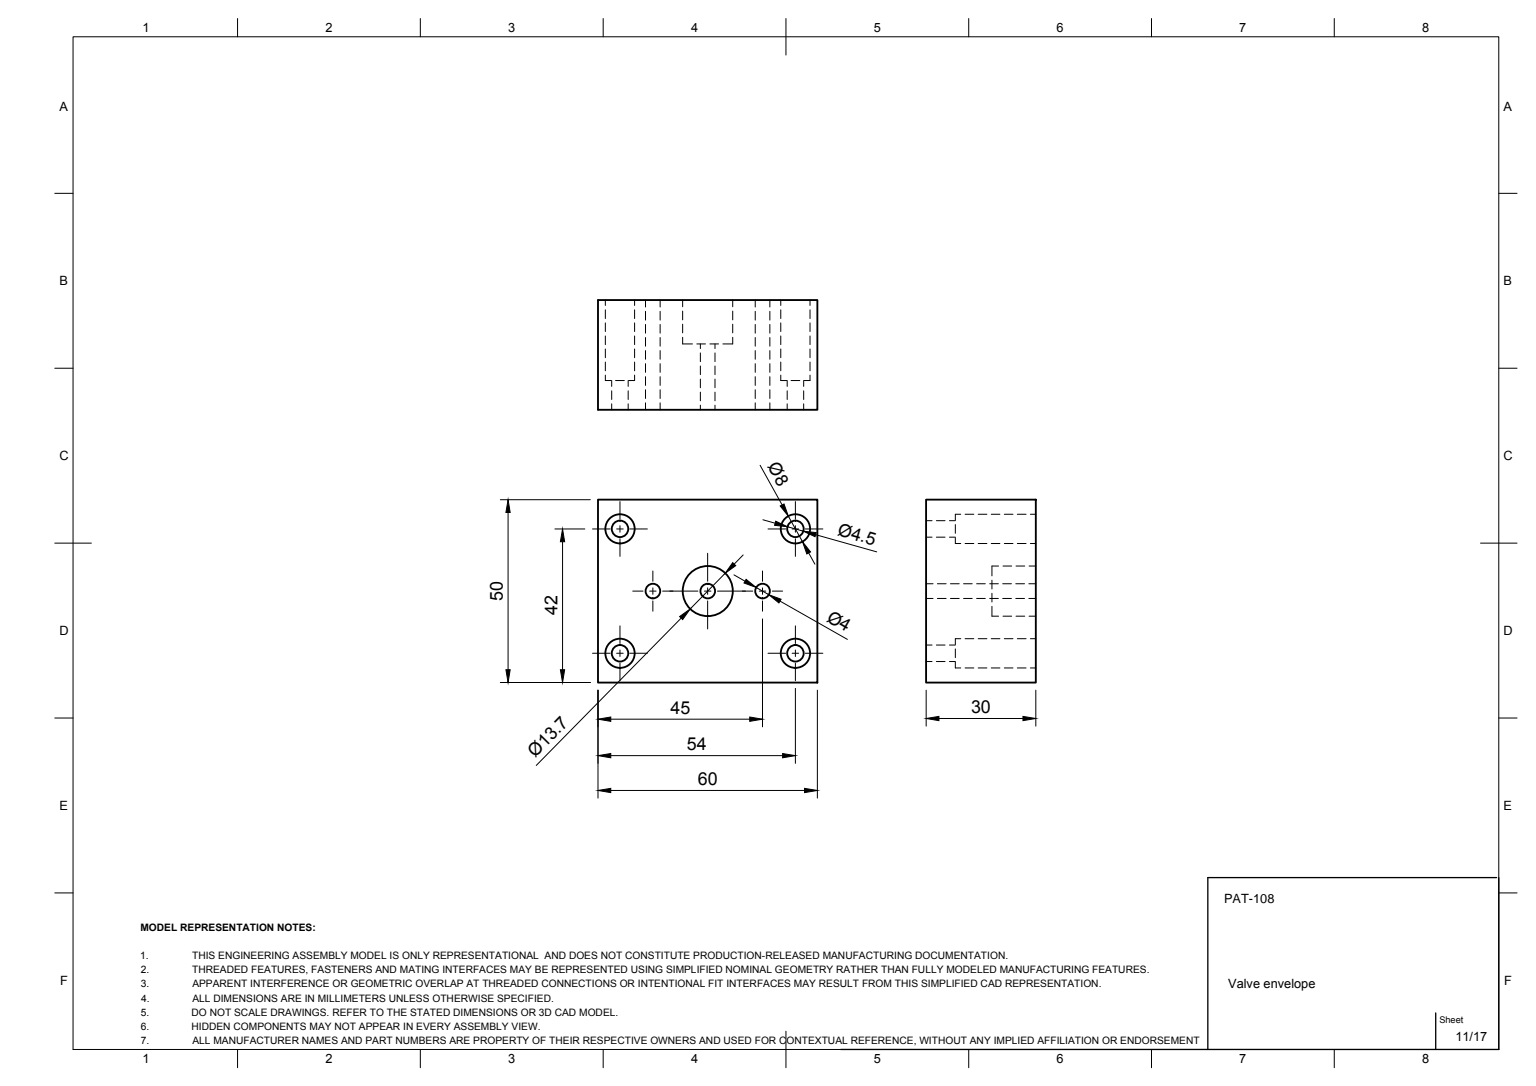
ISO-10303-21;
HEADER;
/* Generated by software containing ST-Developer
 * from STEP Tools, Inc. (www.steptools.com) 
 */

FILE_DESCRIPTION(
/* description */ ('Sub-base valve envelopes and connections'),
/* implementation_level */ '2;1');

FILE_NAME(
/* name */ 'Valve envelope.step',
/* time_stamp */ '2026-10-29T15:55:44-07:00',
/* author */ (''),
/* organization */ (''),
/* preprocessor_version */ 'ST-DEVELOPER v20.2',
/* originating_system */ 'Autodesk Translation Framework v15.17.0.0',
/* authorisation */ '');

FILE_SCHEMA (('AUTOMOTIVE_DESIGN { 1 0 10303 214 3 1 1 }'));
ENDSEC;

DATA;
#10=MECHANICAL_DESIGN_GEOMETRIC_PRESENTATION_REPRESENTATION('',(#125),#6113);
#101=SHAPE_REPRESENTATION_RELATIONSHIP('SRR','None',#6175,#113);
#113=ADVANCED_BREP_SHAPE_REPRESENTATION('',(#137),#6106);
#125=STYLED_ITEM('',(#6301),#137);
#137=MANIFOLD_SOLID_BREP('Body1',#3364);
#212=FACE_BOUND('',#767,.T.);
#213=FACE_BOUND('',#770,.T.);
#214=FACE_BOUND('',#773,.T.);
#215=FACE_BOUND('',#776,.T.);
#216=FACE_BOUND('',#783,.T.);
#217=FACE_BOUND('',#792,.T.);
#218=FACE_BOUND('',#793,.T.);
#219=FACE_BOUND('',#794,.T.);
#220=FACE_BOUND('',#795,.T.);
#221=FACE_BOUND('',#796,.T.);
#222=FACE_BOUND('',#797,.T.);
#223=FACE_BOUND('',#798,.T.);
#224=FACE_BOUND('',#800,.T.);
#225=FACE_BOUND('',#801,.T.);
#226=FACE_BOUND('',#802,.T.);
#227=FACE_BOUND('',#803,.T.);
#228=FACE_BOUND('',#804,.T.);
#229=FACE_BOUND('',#805,.T.);
#230=FACE_BOUND('',#806,.T.);
#333=PLANE('',#3726);
#334=PLANE('',#3731);
#335=PLANE('',#3736);
#336=PLANE('',#3741);
#337=PLANE('',#3754);
#338=PLANE('',#3764);
#339=PLANE('',#3765);
#340=PLANE('',#3766);
#341=PLANE('',#3767);
#342=PLANE('',#3768);
#343=PLANE('',#3769);
#496=FACE_OUTER_BOUND('',#765,.T.);
#497=FACE_OUTER_BOUND('',#766,.T.);
#498=FACE_OUTER_BOUND('',#768,.T.);
#499=FACE_OUTER_BOUND('',#769,.T.);
#500=FACE_OUTER_BOUND('',#771,.T.);
#501=FACE_OUTER_BOUND('',#772,.T.);
#502=FACE_OUTER_BOUND('',#774,.T.);
#503=FACE_OUTER_BOUND('',#775,.T.);
#504=FACE_OUTER_BOUND('',#777,.T.);
#505=FACE_OUTER_BOUND('',#778,.T.);
#506=FACE_OUTER_BOUND('',#779,.T.);
#507=FACE_OUTER_BOUND('',#780,.T.);
#508=FACE_OUTER_BOUND('',#781,.T.);
#509=FACE_OUTER_BOUND('',#782,.T.);
#510=FACE_OUTER_BOUND('',#784,.T.);
#511=FACE_OUTER_BOUND('',#785,.T.);
#512=FACE_OUTER_BOUND('',#786,.T.);
#513=FACE_OUTER_BOUND('',#787,.T.);
#514=FACE_OUTER_BOUND('',#788,.T.);
#515=FACE_OUTER_BOUND('',#789,.T.);
#516=FACE_OUTER_BOUND('',#790,.T.);
#517=FACE_OUTER_BOUND('',#791,.T.);
#518=FACE_OUTER_BOUND('',#799,.T.);
#765=EDGE_LOOP('',(#2711,#2712,#2713,#2714));
#766=EDGE_LOOP('',(#2715));
#767=EDGE_LOOP('',(#2716));
#768=EDGE_LOOP('',(#2717,#2718,#2719,#2720));
#769=EDGE_LOOP('',(#2721));
#770=EDGE_LOOP('',(#2722));
#771=EDGE_LOOP('',(#2723,#2724,#2725,#2726));
#772=EDGE_LOOP('',(#2727));
#773=EDGE_LOOP('',(#2728));
#774=EDGE_LOOP('',(#2729,#2730,#2731,#2732));
#775=EDGE_LOOP('',(#2733));
#776=EDGE_LOOP('',(#2734));
#777=EDGE_LOOP('',(#2735,#2736,#2737,#2738));
#778=EDGE_LOOP('',(#2739,#2740,#2741,#2742));
#779=EDGE_LOOP('',(#2743,#2744,#2745,#2746));
#780=EDGE_LOOP('',(#2747,#2748,#2749,#2750));
#781=EDGE_LOOP('',(#2751,#2752,#2753,#2754));
#782=EDGE_LOOP('',(#2755));
#783=EDGE_LOOP('',(#2756));
#784=EDGE_LOOP('',(#2757,#2758,#2759,#2760));
#785=EDGE_LOOP('',(#2761,#2762,#2763,#2764));
#786=EDGE_LOOP('',(#2765,#2766,#2767,#2768));
#787=EDGE_LOOP('',(#2769,#2770,#2771,#2772));
#788=EDGE_LOOP('',(#2773,#2774,#2775,#2776));
#789=EDGE_LOOP('',(#2777,#2778,#2779,#2780));
#790=EDGE_LOOP('',(#2781,#2782,#2783,#2784));
#791=EDGE_LOOP('',(#2785,#2786,#2787,#2788));
#792=EDGE_LOOP('',(#2789));
#793=EDGE_LOOP('',(#2790));
#794=EDGE_LOOP('',(#2791));
#795=EDGE_LOOP('',(#2792));
#796=EDGE_LOOP('',(#2793));
#797=EDGE_LOOP('',(#2794));
#798=EDGE_LOOP('',(#2795));
#799=EDGE_LOOP('',(#2796,#2797,#2798,#2799));
#800=EDGE_LOOP('',(#2800));
#801=EDGE_LOOP('',(#2801));
#802=EDGE_LOOP('',(#2802));
#803=EDGE_LOOP('',(#2803));
#804=EDGE_LOOP('',(#2804));
#805=EDGE_LOOP('',(#2805));
#806=EDGE_LOOP('',(#2806));
#1021=LINE('',#5670,#1255);
#1022=LINE('',#5679,#1256);
#1023=LINE('',#5688,#1257);
#1024=LINE('',#5697,#1258);
#1025=LINE('',#5705,#1259);
#1026=LINE('',#5709,#1260);
#1027=LINE('',#5713,#1261);
#1028=LINE('',#5717,#1262);
#1029=LINE('',#5722,#1263);
#1030=LINE('',#5731,#1264);
#1031=LINE('',#5736,#1265);
#1032=LINE('',#5741,#1266);
#1033=LINE('',#5746,#1267);
#1034=LINE('',#5748,#1268);
#1035=LINE('',#5750,#1269);
#1036=LINE('',#5751,#1270);
#1037=LINE('',#5754,#1271);
#1038=LINE('',#5756,#1272);
#1039=LINE('',#5757,#1273);
#1040=LINE('',#5760,#1274);
#1041=LINE('',#5762,#1275);
#1042=LINE('',#5763,#1276);
#1043=LINE('',#5765,#1277);
#1044=LINE('',#5766,#1278);
#1255=VECTOR('',#4467,0.4);
#1256=VECTOR('',#4478,0.4);
#1257=VECTOR('',#4489,0.4);
#1258=VECTOR('',#4500,0.4);
#1259=VECTOR('',#4511,0.225);
#1260=VECTOR('',#4516,0.225);
#1261=VECTOR('',#4521,0.225);
#1262=VECTOR('',#4526,0.225);
#1263=VECTOR('',#4531,0.685);
#1264=VECTOR('',#4542,0.2);
#1265=VECTOR('',#4549,0.2);
#1266=VECTOR('',#4554,0.2);
#1267=VECTOR('',#4559,1.);
#1268=VECTOR('',#4560,1.);
#1269=VECTOR('',#4561,1.);
#1270=VECTOR('',#4562,1.);
#1271=VECTOR('',#4565,1.);
#1272=VECTOR('',#4566,1.);
#1273=VECTOR('',#4567,1.);
#1274=VECTOR('',#4570,1.);
#1275=VECTOR('',#4571,1.);
#1276=VECTOR('',#4572,1.);
#1277=VECTOR('',#4575,1.);
#1278=VECTOR('',#4576,1.);
#1469=CIRCLE('',#3724,0.4);
#1470=CIRCLE('',#3725,0.4);
#1471=CIRCLE('',#3727,0.225);
#1472=CIRCLE('',#3729,0.4);
#1473=CIRCLE('',#3730,0.4);
#1474=CIRCLE('',#3732,0.225);
#1475=CIRCLE('',#3734,0.4);
#1476=CIRCLE('',#3735,0.4);
#1477=CIRCLE('',#3737,0.225);
#1478=CIRCLE('',#3739,0.4);
#1479=CIRCLE('',#3740,0.4);
#1480=CIRCLE('',#3742,0.225);
#1481=CIRCLE('',#3744,0.225);
#1482=CIRCLE('',#3746,0.225);
#1483=CIRCLE('',#3748,0.225);
#1484=CIRCLE('',#3750,0.225);
#1485=CIRCLE('',#3752,0.685);
#1486=CIRCLE('',#3753,0.685);
#1487=CIRCLE('',#3755,0.2);
#1488=CIRCLE('',#3757,0.2);
#1489=CIRCLE('',#3758,0.2);
#1490=CIRCLE('',#3760,0.2);
#1491=CIRCLE('',#3762,0.2);
#1492=CIRCLE('',#3763,0.2);
#1695=VERTEX_POINT('',#5667);
#1696=VERTEX_POINT('',#5669);
#1697=VERTEX_POINT('',#5673);
#1698=VERTEX_POINT('',#5676);
#1699=VERTEX_POINT('',#5678);
#1700=VERTEX_POINT('',#5682);
#1701=VERTEX_POINT('',#5685);
#1702=VERTEX_POINT('',#5687);
#1703=VERTEX_POINT('',#5691);
#1704=VERTEX_POINT('',#5694);
#1705=VERTEX_POINT('',#5696);
#1706=VERTEX_POINT('',#5700);
#1707=VERTEX_POINT('',#5703);
#1708=VERTEX_POINT('',#5707);
#1709=VERTEX_POINT('',#5711);
#1710=VERTEX_POINT('',#5715);
#1711=VERTEX_POINT('',#5719);
#1712=VERTEX_POINT('',#5721);
#1713=VERTEX_POINT('',#5725);
#1714=VERTEX_POINT('',#5728);
#1715=VERTEX_POINT('',#5730);
#1716=VERTEX_POINT('',#5734);
#1717=VERTEX_POINT('',#5738);
#1718=VERTEX_POINT('',#5740);
#1719=VERTEX_POINT('',#5744);
#1720=VERTEX_POINT('',#5745);
#1721=VERTEX_POINT('',#5747);
#1722=VERTEX_POINT('',#5749);
#1723=VERTEX_POINT('',#5753);
#1724=VERTEX_POINT('',#5755);
#1725=VERTEX_POINT('',#5759);
#1726=VERTEX_POINT('',#5761);
#2053=EDGE_CURVE('',#1695,#1695,#1469,.T.);
#2054=EDGE_CURVE('',#1695,#1696,#1021,.T.);
#2055=EDGE_CURVE('',#1696,#1696,#1470,.T.);
#2056=EDGE_CURVE('',#1697,#1697,#1471,.T.);
#2057=EDGE_CURVE('',#1698,#1698,#1472,.T.);
#2058=EDGE_CURVE('',#1698,#1699,#1022,.T.);
#2059=EDGE_CURVE('',#1699,#1699,#1473,.T.);
#2060=EDGE_CURVE('',#1700,#1700,#1474,.T.);
#2061=EDGE_CURVE('',#1701,#1701,#1475,.T.);
#2062=EDGE_CURVE('',#1701,#1702,#1023,.T.);
#2063=EDGE_CURVE('',#1702,#1702,#1476,.T.);
#2064=EDGE_CURVE('',#1703,#1703,#1477,.T.);
#2065=EDGE_CURVE('',#1704,#1704,#1478,.T.);
#2066=EDGE_CURVE('',#1704,#1705,#1024,.T.);
#2067=EDGE_CURVE('',#1705,#1705,#1479,.T.);
#2068=EDGE_CURVE('',#1706,#1706,#1480,.T.);
#2069=EDGE_CURVE('',#1707,#1707,#1481,.T.);
#2070=EDGE_CURVE('',#1707,#1697,#1025,.T.);
#2071=EDGE_CURVE('',#1708,#1708,#1482,.T.);
#2072=EDGE_CURVE('',#1708,#1700,#1026,.T.);
#2073=EDGE_CURVE('',#1709,#1709,#1483,.T.);
#2074=EDGE_CURVE('',#1709,#1703,#1027,.T.);
#2075=EDGE_CURVE('',#1710,#1710,#1484,.T.);
#2076=EDGE_CURVE('',#1710,#1706,#1028,.T.);
#2077=EDGE_CURVE('',#1711,#1711,#1485,.T.);
#2078=EDGE_CURVE('',#1711,#1712,#1029,.T.);
#2079=EDGE_CURVE('',#1712,#1712,#1486,.T.);
#2080=EDGE_CURVE('',#1713,#1713,#1487,.T.);
#2081=EDGE_CURVE('',#1714,#1714,#1488,.T.);
#2082=EDGE_CURVE('',#1714,#1715,#1030,.T.);
#2083=EDGE_CURVE('',#1715,#1715,#1489,.T.);
#2084=EDGE_CURVE('',#1716,#1716,#1490,.T.);
#2085=EDGE_CURVE('',#1716,#1713,#1031,.T.);
#2086=EDGE_CURVE('',#1717,#1717,#1491,.T.);
#2087=EDGE_CURVE('',#1717,#1718,#1032,.T.);
#2088=EDGE_CURVE('',#1718,#1718,#1492,.T.);
#2089=EDGE_CURVE('',#1719,#1720,#1033,.T.);
#2090=EDGE_CURVE('',#1720,#1721,#1034,.T.);
#2091=EDGE_CURVE('',#1722,#1721,#1035,.T.);
#2092=EDGE_CURVE('',#1719,#1722,#1036,.T.);
#2093=EDGE_CURVE('',#1723,#1719,#1037,.T.);
#2094=EDGE_CURVE('',#1724,#1722,#1038,.T.);
#2095=EDGE_CURVE('',#1723,#1724,#1039,.T.);
#2096=EDGE_CURVE('',#1725,#1723,#1040,.T.);
#2097=EDGE_CURVE('',#1726,#1724,#1041,.T.);
#2098=EDGE_CURVE('',#1725,#1726,#1042,.T.);
#2099=EDGE_CURVE('',#1720,#1725,#1043,.T.);
#2100=EDGE_CURVE('',#1721,#1726,#1044,.T.);
#2711=ORIENTED_EDGE('',*,*,#2053,.F.);
#2712=ORIENTED_EDGE('',*,*,#2054,.T.);
#2713=ORIENTED_EDGE('',*,*,#2055,.F.);
#2714=ORIENTED_EDGE('',*,*,#2054,.F.);
#2715=ORIENTED_EDGE('',*,*,#2053,.T.);
#2716=ORIENTED_EDGE('',*,*,#2056,.F.);
#2717=ORIENTED_EDGE('',*,*,#2057,.F.);
#2718=ORIENTED_EDGE('',*,*,#2058,.T.);
#2719=ORIENTED_EDGE('',*,*,#2059,.F.);
#2720=ORIENTED_EDGE('',*,*,#2058,.F.);
#2721=ORIENTED_EDGE('',*,*,#2057,.T.);
#2722=ORIENTED_EDGE('',*,*,#2060,.F.);
#2723=ORIENTED_EDGE('',*,*,#2061,.F.);
#2724=ORIENTED_EDGE('',*,*,#2062,.T.);
#2725=ORIENTED_EDGE('',*,*,#2063,.F.);
#2726=ORIENTED_EDGE('',*,*,#2062,.F.);
#2727=ORIENTED_EDGE('',*,*,#2061,.T.);
#2728=ORIENTED_EDGE('',*,*,#2064,.F.);
#2729=ORIENTED_EDGE('',*,*,#2065,.F.);
#2730=ORIENTED_EDGE('',*,*,#2066,.T.);
#2731=ORIENTED_EDGE('',*,*,#2067,.F.);
#2732=ORIENTED_EDGE('',*,*,#2066,.F.);
#2733=ORIENTED_EDGE('',*,*,#2065,.T.);
#2734=ORIENTED_EDGE('',*,*,#2068,.F.);
#2735=ORIENTED_EDGE('',*,*,#2069,.F.);
#2736=ORIENTED_EDGE('',*,*,#2070,.T.);
#2737=ORIENTED_EDGE('',*,*,#2056,.T.);
#2738=ORIENTED_EDGE('',*,*,#2070,.F.);
#2739=ORIENTED_EDGE('',*,*,#2071,.F.);
#2740=ORIENTED_EDGE('',*,*,#2072,.T.);
#2741=ORIENTED_EDGE('',*,*,#2060,.T.);
#2742=ORIENTED_EDGE('',*,*,#2072,.F.);
#2743=ORIENTED_EDGE('',*,*,#2073,.F.);
#2744=ORIENTED_EDGE('',*,*,#2074,.T.);
#2745=ORIENTED_EDGE('',*,*,#2064,.T.);
#2746=ORIENTED_EDGE('',*,*,#2074,.F.);
#2747=ORIENTED_EDGE('',*,*,#2075,.F.);
#2748=ORIENTED_EDGE('',*,*,#2076,.T.);
#2749=ORIENTED_EDGE('',*,*,#2068,.T.);
#2750=ORIENTED_EDGE('',*,*,#2076,.F.);
#2751=ORIENTED_EDGE('',*,*,#2077,.F.);
#2752=ORIENTED_EDGE('',*,*,#2078,.T.);
#2753=ORIENTED_EDGE('',*,*,#2079,.F.);
#2754=ORIENTED_EDGE('',*,*,#2078,.F.);
#2755=ORIENTED_EDGE('',*,*,#2077,.T.);
#2756=ORIENTED_EDGE('',*,*,#2080,.F.);
#2757=ORIENTED_EDGE('',*,*,#2081,.F.);
#2758=ORIENTED_EDGE('',*,*,#2082,.T.);
#2759=ORIENTED_EDGE('',*,*,#2083,.F.);
#2760=ORIENTED_EDGE('',*,*,#2082,.F.);
#2761=ORIENTED_EDGE('',*,*,#2084,.F.);
#2762=ORIENTED_EDGE('',*,*,#2085,.T.);
#2763=ORIENTED_EDGE('',*,*,#2080,.T.);
#2764=ORIENTED_EDGE('',*,*,#2085,.F.);
#2765=ORIENTED_EDGE('',*,*,#2086,.F.);
#2766=ORIENTED_EDGE('',*,*,#2087,.T.);
#2767=ORIENTED_EDGE('',*,*,#2088,.F.);
#2768=ORIENTED_EDGE('',*,*,#2087,.F.);
#2769=ORIENTED_EDGE('',*,*,#2089,.T.);
#2770=ORIENTED_EDGE('',*,*,#2090,.T.);
#2771=ORIENTED_EDGE('',*,*,#2091,.F.);
#2772=ORIENTED_EDGE('',*,*,#2092,.F.);
#2773=ORIENTED_EDGE('',*,*,#2093,.T.);
#2774=ORIENTED_EDGE('',*,*,#2092,.T.);
#2775=ORIENTED_EDGE('',*,*,#2094,.F.);
#2776=ORIENTED_EDGE('',*,*,#2095,.F.);
#2777=ORIENTED_EDGE('',*,*,#2096,.T.);
#2778=ORIENTED_EDGE('',*,*,#2095,.T.);
#2779=ORIENTED_EDGE('',*,*,#2097,.F.);
#2780=ORIENTED_EDGE('',*,*,#2098,.F.);
#2781=ORIENTED_EDGE('',*,*,#2099,.T.);
#2782=ORIENTED_EDGE('',*,*,#2098,.T.);
#2783=ORIENTED_EDGE('',*,*,#2100,.F.);
#2784=ORIENTED_EDGE('',*,*,#2090,.F.);
#2785=ORIENTED_EDGE('',*,*,#2100,.T.);
#2786=ORIENTED_EDGE('',*,*,#2097,.T.);
#2787=ORIENTED_EDGE('',*,*,#2094,.T.);
#2788=ORIENTED_EDGE('',*,*,#2091,.T.);
#2789=ORIENTED_EDGE('',*,*,#2079,.T.);
#2790=ORIENTED_EDGE('',*,*,#2083,.T.);
#2791=ORIENTED_EDGE('',*,*,#2088,.T.);
#2792=ORIENTED_EDGE('',*,*,#2067,.T.);
#2793=ORIENTED_EDGE('',*,*,#2063,.T.);
#2794=ORIENTED_EDGE('',*,*,#2059,.T.);
#2795=ORIENTED_EDGE('',*,*,#2055,.T.);
#2796=ORIENTED_EDGE('',*,*,#2099,.F.);
#2797=ORIENTED_EDGE('',*,*,#2089,.F.);
#2798=ORIENTED_EDGE('',*,*,#2093,.F.);
#2799=ORIENTED_EDGE('',*,*,#2096,.F.);
#2800=ORIENTED_EDGE('',*,*,#2086,.T.);
#2801=ORIENTED_EDGE('',*,*,#2084,.T.);
#2802=ORIENTED_EDGE('',*,*,#2081,.T.);
#2803=ORIENTED_EDGE('',*,*,#2075,.T.);
#2804=ORIENTED_EDGE('',*,*,#2073,.T.);
#2805=ORIENTED_EDGE('',*,*,#2071,.T.);
#2806=ORIENTED_EDGE('',*,*,#2069,.T.);
#3127=CYLINDRICAL_SURFACE('',#3723,0.4);
#3128=CYLINDRICAL_SURFACE('',#3728,0.4);
#3129=CYLINDRICAL_SURFACE('',#3733,0.4);
#3130=CYLINDRICAL_SURFACE('',#3738,0.4);
#3131=CYLINDRICAL_SURFACE('',#3743,0.225);
#3132=CYLINDRICAL_SURFACE('',#3745,0.225);
#3133=CYLINDRICAL_SURFACE('',#3747,0.225);
#3134=CYLINDRICAL_SURFACE('',#3749,0.225);
#3135=CYLINDRICAL_SURFACE('',#3751,0.685);
#3136=CYLINDRICAL_SURFACE('',#3756,0.2);
#3137=CYLINDRICAL_SURFACE('',#3759,0.2);
#3138=CYLINDRICAL_SURFACE('',#3761,0.2);
#3269=ADVANCED_FACE('',(#496),#3127,.F.);
#3270=ADVANCED_FACE('',(#497,#212),#333,.T.);
#3271=ADVANCED_FACE('',(#498),#3128,.F.);
#3272=ADVANCED_FACE('',(#499,#213),#334,.T.);
#3273=ADVANCED_FACE('',(#500),#3129,.F.);
#3274=ADVANCED_FACE('',(#501,#214),#335,.T.);
#3275=ADVANCED_FACE('',(#502),#3130,.F.);
#3276=ADVANCED_FACE('',(#503,#215),#336,.T.);
#3277=ADVANCED_FACE('',(#504),#3131,.F.);
#3278=ADVANCED_FACE('',(#505),#3132,.F.);
#3279=ADVANCED_FACE('',(#506),#3133,.F.);
#3280=ADVANCED_FACE('',(#507),#3134,.F.);
#3281=ADVANCED_FACE('',(#508),#3135,.F.);
#3282=ADVANCED_FACE('',(#509,#216),#337,.T.);
#3283=ADVANCED_FACE('',(#510),#3136,.F.);
#3284=ADVANCED_FACE('',(#511),#3137,.F.);
#3285=ADVANCED_FACE('',(#512),#3138,.F.);
#3286=ADVANCED_FACE('',(#513),#338,.T.);
#3287=ADVANCED_FACE('',(#514),#339,.T.);
#3288=ADVANCED_FACE('',(#515),#340,.T.);
#3289=ADVANCED_FACE('',(#516),#341,.T.);
#3290=ADVANCED_FACE('',(#517,#217,#218,#219,#220,#221,#222,#223),#342,.T.);
#3291=ADVANCED_FACE('',(#518,#224,#225,#226,#227,#228,#229,#230),#343,.F.);
#3364=CLOSED_SHELL('',(#3269,#3270,#3271,#3272,#3273,#3274,#3275,#3276,
#3277,#3278,#3279,#3280,#3281,#3282,#3283,#3284,#3285,#3286,#3287,#3288,
#3289,#3290,#3291));
#3722=AXIS2_PLACEMENT_3D('',#5665,#4461,#4462);
#3723=AXIS2_PLACEMENT_3D('',#5666,#4463,#4464);
#3724=AXIS2_PLACEMENT_3D('',#5668,#4465,#4466);
#3725=AXIS2_PLACEMENT_3D('',#5671,#4468,#4469);
#3726=AXIS2_PLACEMENT_3D('',#5672,#4470,#4471);
#3727=AXIS2_PLACEMENT_3D('',#5674,#4472,#4473);
#3728=AXIS2_PLACEMENT_3D('',#5675,#4474,#4475);
#3729=AXIS2_PLACEMENT_3D('',#5677,#4476,#4477);
#3730=AXIS2_PLACEMENT_3D('',#5680,#4479,#4480);
#3731=AXIS2_PLACEMENT_3D('',#5681,#4481,#4482);
#3732=AXIS2_PLACEMENT_3D('',#5683,#4483,#4484);
#3733=AXIS2_PLACEMENT_3D('',#5684,#4485,#4486);
#3734=AXIS2_PLACEMENT_3D('',#5686,#4487,#4488);
#3735=AXIS2_PLACEMENT_3D('',#5689,#4490,#4491);
#3736=AXIS2_PLACEMENT_3D('',#5690,#4492,#4493);
#3737=AXIS2_PLACEMENT_3D('',#5692,#4494,#4495);
#3738=AXIS2_PLACEMENT_3D('',#5693,#4496,#4497);
#3739=AXIS2_PLACEMENT_3D('',#5695,#4498,#4499);
#3740=AXIS2_PLACEMENT_3D('',#5698,#4501,#4502);
#3741=AXIS2_PLACEMENT_3D('',#5699,#4503,#4504);
#3742=AXIS2_PLACEMENT_3D('',#5701,#4505,#4506);
#3743=AXIS2_PLACEMENT_3D('',#5702,#4507,#4508);
#3744=AXIS2_PLACEMENT_3D('',#5704,#4509,#4510);
#3745=AXIS2_PLACEMENT_3D('',#5706,#4512,#4513);
#3746=AXIS2_PLACEMENT_3D('',#5708,#4514,#4515);
#3747=AXIS2_PLACEMENT_3D('',#5710,#4517,#4518);
#3748=AXIS2_PLACEMENT_3D('',#5712,#4519,#4520);
#3749=AXIS2_PLACEMENT_3D('',#5714,#4522,#4523);
#3750=AXIS2_PLACEMENT_3D('',#5716,#4524,#4525);
#3751=AXIS2_PLACEMENT_3D('',#5718,#4527,#4528);
#3752=AXIS2_PLACEMENT_3D('',#5720,#4529,#4530);
#3753=AXIS2_PLACEMENT_3D('',#5723,#4532,#4533);
#3754=AXIS2_PLACEMENT_3D('',#5724,#4534,#4535);
#3755=AXIS2_PLACEMENT_3D('',#5726,#4536,#4537);
#3756=AXIS2_PLACEMENT_3D('',#5727,#4538,#4539);
#3757=AXIS2_PLACEMENT_3D('',#5729,#4540,#4541);
#3758=AXIS2_PLACEMENT_3D('',#5732,#4543,#4544);
#3759=AXIS2_PLACEMENT_3D('',#5733,#4545,#4546);
#3760=AXIS2_PLACEMENT_3D('',#5735,#4547,#4548);
#3761=AXIS2_PLACEMENT_3D('',#5737,#4550,#4551);
#3762=AXIS2_PLACEMENT_3D('',#5739,#4552,#4553);
#3763=AXIS2_PLACEMENT_3D('',#5742,#4555,#4556);
#3764=AXIS2_PLACEMENT_3D('',#5743,#4557,#4558);
#3765=AXIS2_PLACEMENT_3D('',#5752,#4563,#4564);
#3766=AXIS2_PLACEMENT_3D('',#5758,#4568,#4569);
#3767=AXIS2_PLACEMENT_3D('',#5764,#4573,#4574);
#3768=AXIS2_PLACEMENT_3D('',#5767,#4577,#4578);
#3769=AXIS2_PLACEMENT_3D('',#5768,#4579,#4580);
#4461=DIRECTION('axis',(0.,0.,1.));
#4462=DIRECTION('refdir',(1.,0.,0.));
#4463=DIRECTION('center_axis',(0.,0.,1.));
#4464=DIRECTION('ref_axis',(1.,0.,0.));
#4465=DIRECTION('center_axis',(0.,0.,1.));
#4466=DIRECTION('ref_axis',(1.,0.,0.));
#4467=DIRECTION('',(0.,0.,1.));
#4468=DIRECTION('center_axis',(0.,0.,-1.));
#4469=DIRECTION('ref_axis',(1.,0.,0.));
#4470=DIRECTION('center_axis',(0.,0.,1.));
#4471=DIRECTION('ref_axis',(1.,0.,0.));
#4472=DIRECTION('center_axis',(0.,0.,1.));
#4473=DIRECTION('ref_axis',(1.,0.,0.));
#4474=DIRECTION('center_axis',(0.,0.,1.));
#4475=DIRECTION('ref_axis',(1.,0.,0.));
#4476=DIRECTION('center_axis',(0.,0.,1.));
#4477=DIRECTION('ref_axis',(1.,0.,0.));
#4478=DIRECTION('',(0.,0.,1.));
#4479=DIRECTION('center_axis',(0.,0.,-1.));
#4480=DIRECTION('ref_axis',(1.,0.,0.));
#4481=DIRECTION('center_axis',(0.,0.,1.));
#4482=DIRECTION('ref_axis',(1.,0.,0.));
#4483=DIRECTION('center_axis',(0.,0.,1.));
#4484=DIRECTION('ref_axis',(1.,0.,0.));
#4485=DIRECTION('center_axis',(0.,0.,1.));
#4486=DIRECTION('ref_axis',(1.,0.,0.));
#4487=DIRECTION('center_axis',(0.,0.,1.));
#4488=DIRECTION('ref_axis',(1.,0.,0.));
#4489=DIRECTION('',(0.,0.,1.));
#4490=DIRECTION('center_axis',(0.,0.,-1.));
#4491=DIRECTION('ref_axis',(1.,0.,0.));
#4492=DIRECTION('center_axis',(0.,0.,1.));
#4493=DIRECTION('ref_axis',(1.,0.,0.));
#4494=DIRECTION('center_axis',(0.,0.,1.));
#4495=DIRECTION('ref_axis',(1.,0.,0.));
#4496=DIRECTION('center_axis',(0.,0.,1.));
#4497=DIRECTION('ref_axis',(1.,0.,0.));
#4498=DIRECTION('center_axis',(0.,0.,1.));
#4499=DIRECTION('ref_axis',(1.,0.,0.));
#4500=DIRECTION('',(0.,0.,1.));
#4501=DIRECTION('center_axis',(0.,0.,-1.));
#4502=DIRECTION('ref_axis',(1.,0.,0.));
#4503=DIRECTION('center_axis',(0.,0.,1.));
#4504=DIRECTION('ref_axis',(1.,0.,0.));
#4505=DIRECTION('center_axis',(0.,0.,1.));
#4506=DIRECTION('ref_axis',(1.,0.,0.));
#4507=DIRECTION('center_axis',(0.,0.,1.));
#4508=DIRECTION('ref_axis',(1.,0.,0.));
#4509=DIRECTION('center_axis',(0.,0.,1.));
#4510=DIRECTION('ref_axis',(1.,0.,0.));
#4511=DIRECTION('',(0.,0.,1.));
#4512=DIRECTION('center_axis',(0.,0.,1.));
#4513=DIRECTION('ref_axis',(1.,0.,0.));
#4514=DIRECTION('center_axis',(0.,0.,1.));
#4515=DIRECTION('ref_axis',(1.,0.,0.));
#4516=DIRECTION('',(0.,0.,1.));
#4517=DIRECTION('center_axis',(0.,0.,1.));
#4518=DIRECTION('ref_axis',(1.,0.,0.));
#4519=DIRECTION('center_axis',(0.,0.,1.));
#4520=DIRECTION('ref_axis',(1.,0.,0.));
#4521=DIRECTION('',(0.,0.,1.));
#4522=DIRECTION('center_axis',(0.,0.,1.));
#4523=DIRECTION('ref_axis',(1.,0.,0.));
#4524=DIRECTION('center_axis',(0.,0.,1.));
#4525=DIRECTION('ref_axis',(1.,0.,0.));
#4526=DIRECTION('',(0.,0.,1.));
#4527=DIRECTION('center_axis',(0.,0.,1.));
#4528=DIRECTION('ref_axis',(1.,0.,0.));
#4529=DIRECTION('center_axis',(0.,0.,1.));
#4530=DIRECTION('ref_axis',(1.,0.,0.));
#4531=DIRECTION('',(0.,0.,1.));
#4532=DIRECTION('center_axis',(0.,0.,-1.));
#4533=DIRECTION('ref_axis',(1.,0.,0.));
#4534=DIRECTION('center_axis',(0.,0.,1.));
#4535=DIRECTION('ref_axis',(1.,0.,0.));
#4536=DIRECTION('center_axis',(0.,0.,1.));
#4537=DIRECTION('ref_axis',(1.,0.,0.));
#4538=DIRECTION('center_axis',(0.,0.,1.));
#4539=DIRECTION('ref_axis',(1.,0.,0.));
#4540=DIRECTION('center_axis',(0.,0.,1.));
#4541=DIRECTION('ref_axis',(1.,0.,0.));
#4542=DIRECTION('',(0.,0.,1.));
#4543=DIRECTION('center_axis',(0.,0.,-1.));
#4544=DIRECTION('ref_axis',(1.,0.,0.));
#4545=DIRECTION('center_axis',(0.,0.,1.));
#4546=DIRECTION('ref_axis',(1.,0.,0.));
#4547=DIRECTION('center_axis',(0.,0.,1.));
#4548=DIRECTION('ref_axis',(1.,0.,0.));
#4549=DIRECTION('',(0.,0.,1.));
#4550=DIRECTION('center_axis',(0.,0.,1.));
#4551=DIRECTION('ref_axis',(1.,0.,0.));
#4552=DIRECTION('center_axis',(0.,0.,1.));
#4553=DIRECTION('ref_axis',(1.,0.,0.));
#4554=DIRECTION('',(0.,0.,1.));
#4555=DIRECTION('center_axis',(0.,0.,-1.));
#4556=DIRECTION('ref_axis',(1.,0.,0.));
#4557=DIRECTION('center_axis',(0.,1.,0.));
#4558=DIRECTION('ref_axis',(-1.,0.,0.));
#4559=DIRECTION('',(-1.,0.,0.));
#4560=DIRECTION('',(0.,0.,1.));
#4561=DIRECTION('',(-1.,0.,0.));
#4562=DIRECTION('',(0.,0.,1.));
#4563=DIRECTION('center_axis',(1.,0.,0.));
#4564=DIRECTION('ref_axis',(0.,1.,0.));
#4565=DIRECTION('',(0.,1.,0.));
#4566=DIRECTION('',(0.,1.,0.));
#4567=DIRECTION('',(0.,0.,1.));
#4568=DIRECTION('center_axis',(0.,-1.,0.));
#4569=DIRECTION('ref_axis',(1.,0.,0.));
#4570=DIRECTION('',(1.,0.,0.));
#4571=DIRECTION('',(1.,0.,0.));
#4572=DIRECTION('',(0.,0.,1.));
#4573=DIRECTION('center_axis',(-1.,0.,0.));
#4574=DIRECTION('ref_axis',(0.,-1.,0.));
#4575=DIRECTION('',(0.,-1.,0.));
#4576=DIRECTION('',(0.,-1.,0.));
#4577=DIRECTION('center_axis',(0.,0.,1.));
#4578=DIRECTION('ref_axis',(1.,0.,0.));
#4579=DIRECTION('center_axis',(0.,0.,1.));
#4580=DIRECTION('ref_axis',(1.,0.,0.));
#5665=CARTESIAN_POINT('',(0.,0.,0.));
#5666=CARTESIAN_POINT('Origin',(-2.3,-2.4,3.));
#5667=CARTESIAN_POINT('',(-2.7,-2.4,3.));
#5668=CARTESIAN_POINT('Origin',(-2.3,-2.4,3.));
#5669=CARTESIAN_POINT('',(-2.7,-2.4,5.2));
#5670=CARTESIAN_POINT('',(-2.7,-2.4,3.));
#5671=CARTESIAN_POINT('Origin',(-2.3,-2.4,5.2));
#5672=CARTESIAN_POINT('Origin',(-2.3,-2.4,3.));
#5673=CARTESIAN_POINT('',(-2.525,-2.4,3.));
#5674=CARTESIAN_POINT('Origin',(-2.3,-2.4,3.));
#5675=CARTESIAN_POINT('Origin',(-5.7,2.4,3.));
#5676=CARTESIAN_POINT('',(-6.1,2.4,3.));
#5677=CARTESIAN_POINT('Origin',(-5.7,2.4,3.));
#5678=CARTESIAN_POINT('',(-6.1,2.4,5.2));
#5679=CARTESIAN_POINT('',(-6.1,2.4,3.));
#5680=CARTESIAN_POINT('Origin',(-5.7,2.4,5.2));
#5681=CARTESIAN_POINT('Origin',(-5.7,2.4,3.));
#5682=CARTESIAN_POINT('',(-5.925,2.4,3.));
#5683=CARTESIAN_POINT('Origin',(-5.7,2.4,3.));
#5684=CARTESIAN_POINT('Origin',(-5.7,-2.4,3.));
#5685=CARTESIAN_POINT('',(-6.1,-2.4,3.));
#5686=CARTESIAN_POINT('Origin',(-5.7,-2.4,3.));
#5687=CARTESIAN_POINT('',(-6.1,-2.4,5.2));
#5688=CARTESIAN_POINT('',(-6.1,-2.4,3.));
#5689=CARTESIAN_POINT('Origin',(-5.7,-2.4,5.2));
#5690=CARTESIAN_POINT('Origin',(-5.7,-2.4,3.));
#5691=CARTESIAN_POINT('',(-5.925,-2.4,3.));
#5692=CARTESIAN_POINT('Origin',(-5.7,-2.4,3.));
#5693=CARTESIAN_POINT('Origin',(-2.3,2.4,3.));
#5694=CARTESIAN_POINT('',(-2.7,2.4,3.));
#5695=CARTESIAN_POINT('Origin',(-2.3,2.4,3.));
#5696=CARTESIAN_POINT('',(-2.7,2.4,5.2));
#5697=CARTESIAN_POINT('',(-2.7,2.4,3.));
#5698=CARTESIAN_POINT('Origin',(-2.3,2.4,5.2));
#5699=CARTESIAN_POINT('Origin',(-2.3,2.4,3.));
#5700=CARTESIAN_POINT('',(-2.525,2.4,3.));
#5701=CARTESIAN_POINT('Origin',(-2.3,2.4,3.));
#5702=CARTESIAN_POINT('Origin',(-2.3,-2.4,2.1));
#5703=CARTESIAN_POINT('',(-2.525,-2.4,2.2));
#5704=CARTESIAN_POINT('Origin',(-2.3,-2.4,2.2));
#5705=CARTESIAN_POINT('',(-2.525,-2.4,2.1));
#5706=CARTESIAN_POINT('Origin',(-5.7,2.4,2.1));
#5707=CARTESIAN_POINT('',(-5.925,2.4,2.2));
#5708=CARTESIAN_POINT('Origin',(-5.7,2.4,2.2));
#5709=CARTESIAN_POINT('',(-5.925,2.4,2.1));
#5710=CARTESIAN_POINT('Origin',(-5.7,-2.4,2.1));
#5711=CARTESIAN_POINT('',(-5.925,-2.4,2.2));
#5712=CARTESIAN_POINT('Origin',(-5.7,-2.4,2.2));
#5713=CARTESIAN_POINT('',(-5.925,-2.4,2.1));
#5714=CARTESIAN_POINT('Origin',(-2.3,2.4,2.1));
#5715=CARTESIAN_POINT('',(-2.525,2.4,2.2));
#5716=CARTESIAN_POINT('Origin',(-2.3,2.4,2.2));
#5717=CARTESIAN_POINT('',(-2.525,2.4,2.1));
#5718=CARTESIAN_POINT('Origin',(-4.,0.,4.));
#5719=CARTESIAN_POINT('',(-4.685,-8.38883057415937E-17,4.));
#5720=CARTESIAN_POINT('Origin',(-4.,0.,4.));
#5721=CARTESIAN_POINT('',(-4.685,8.38883057415937E-17,5.2));
#5722=CARTESIAN_POINT('',(-4.685,-8.38883057415937E-17,4.));
#5723=CARTESIAN_POINT('Origin',(-4.,0.,5.2));
#5724=CARTESIAN_POINT('Origin',(-4.,0.,4.));
#5725=CARTESIAN_POINT('',(-4.2,-2.44929359829471E-17,4.));
#5726=CARTESIAN_POINT('Origin',(-4.,0.,4.));
#5727=CARTESIAN_POINT('Origin',(-4.,-1.5,2.1));
#5728=CARTESIAN_POINT('',(-4.2,-1.5,2.2));
#5729=CARTESIAN_POINT('Origin',(-4.,-1.5,2.2));
#5730=CARTESIAN_POINT('',(-4.2,-1.5,5.2));
#5731=CARTESIAN_POINT('',(-4.2,-1.5,2.1));
#5732=CARTESIAN_POINT('Origin',(-4.,-1.5,5.2));
#5733=CARTESIAN_POINT('Origin',(-4.,0.,2.1));
#5734=CARTESIAN_POINT('',(-4.2,-2.44929359829471E-17,2.2));
#5735=CARTESIAN_POINT('Origin',(-4.,0.,2.2));
#5736=CARTESIAN_POINT('',(-4.2,-2.44929359829471E-17,2.1));
#5737=CARTESIAN_POINT('Origin',(-4.,1.5,2.1));
#5738=CARTESIAN_POINT('',(-4.2,1.5,2.2));
#5739=CARTESIAN_POINT('Origin',(-4.,1.5,2.2));
#5740=CARTESIAN_POINT('',(-4.2,1.5,5.2));
#5741=CARTESIAN_POINT('',(-4.2,1.5,2.1));
#5742=CARTESIAN_POINT('Origin',(-4.,1.5,5.2));
#5743=CARTESIAN_POINT('Origin',(-1.5,3.,2.2));
#5744=CARTESIAN_POINT('',(-1.5,3.,2.2));
#5745=CARTESIAN_POINT('',(-6.5,3.,2.2));
#5746=CARTESIAN_POINT('',(-1.5,3.,2.2));
#5747=CARTESIAN_POINT('',(-6.5,3.,5.2));
#5748=CARTESIAN_POINT('',(-6.5,3.,2.2));
#5749=CARTESIAN_POINT('',(-1.5,3.,5.2));
#5750=CARTESIAN_POINT('',(-1.5,3.,5.2));
#5751=CARTESIAN_POINT('',(-1.5,3.,2.2));
#5752=CARTESIAN_POINT('Origin',(-1.5,-3.,2.2));
#5753=CARTESIAN_POINT('',(-1.5,-3.,2.2));
#5754=CARTESIAN_POINT('',(-1.5,-3.,2.2));
#5755=CARTESIAN_POINT('',(-1.5,-3.,5.2));
#5756=CARTESIAN_POINT('',(-1.5,-3.,5.2));
#5757=CARTESIAN_POINT('',(-1.5,-3.,2.2));
#5758=CARTESIAN_POINT('Origin',(-6.5,-3.,2.2));
#5759=CARTESIAN_POINT('',(-6.5,-3.,2.2));
#5760=CARTESIAN_POINT('',(-6.5,-3.,2.2));
#5761=CARTESIAN_POINT('',(-6.5,-3.,5.2));
#5762=CARTESIAN_POINT('',(-6.5,-3.,5.2));
#5763=CARTESIAN_POINT('',(-6.5,-3.,2.2));
#5764=CARTESIAN_POINT('Origin',(-6.5,3.,2.2));
#5765=CARTESIAN_POINT('',(-6.5,3.,2.2));
#5766=CARTESIAN_POINT('',(-6.5,3.,5.2));
#5767=CARTESIAN_POINT('Origin',(-4.,0.,5.2));
#5768=CARTESIAN_POINT('Origin',(-4.,0.,2.2));
#6090=UNCERTAINTY_MEASURE_WITH_UNIT(LENGTH_MEASURE(0.001),#6114,
'DISTANCE_ACCURACY_VALUE',
'Maximum model space distance between geometric entities at asserted c
onnectivities');
#6097=UNCERTAINTY_MEASURE_WITH_UNIT(LENGTH_MEASURE(0.001),#6114,
'DISTANCE_ACCURACY_VALUE',
'Maximum model space distance between geometric entities at asserted c
onnectivities');
#6106=(
GEOMETRIC_REPRESENTATION_CONTEXT(3)
GLOBAL_UNCERTAINTY_ASSIGNED_CONTEXT((#6090))
GLOBAL_UNIT_ASSIGNED_CONTEXT((#6114,#6116,#6117))
REPRESENTATION_CONTEXT('','3D')
);
#6113=(
GEOMETRIC_REPRESENTATION_CONTEXT(3)
GLOBAL_UNCERTAINTY_ASSIGNED_CONTEXT((#6097))
GLOBAL_UNIT_ASSIGNED_CONTEXT((#6114,#6116,#6117))
REPRESENTATION_CONTEXT('','3D')
);
#6114=(
LENGTH_UNIT()
NAMED_UNIT(*)
SI_UNIT(.CENTI.,.METRE.)
);
#6116=(
NAMED_UNIT(*)
PLANE_ANGLE_UNIT()
SI_UNIT($,.RADIAN.)
);
#6117=(
NAMED_UNIT(*)
SI_UNIT($,.STERADIAN.)
SOLID_ANGLE_UNIT()
);
#6126=SHAPE_DEFINITION_REPRESENTATION(#6141,#6175);
#6141=PRODUCT_DEFINITION_SHAPE('',$,#6191);
#6175=SHAPE_REPRESENTATION('',(#3722),#6106);
#6182=PRODUCT_DEFINITION_CONTEXT('part definition',#6229,'design');
#6191=PRODUCT_DEFINITION('Valve envelope','Valve envelope',#6206,
#6182);
#6206=PRODUCT_DEFINITION_FORMATION('',$,#6239);
#6229=APPLICATION_CONTEXT(
'Core Data for Automotive Mechanical Design Process');
#6230=PRODUCT_CONTEXT('part definition',#6229,'mechanical');
#6239=PRODUCT('Valve envelope','Valve envelope',
'Valve envelope',(#6230));
#6295=COLOUR_RGB('Light Blue',0.38,0.62,0.78);
#6296=FILL_AREA_STYLE_COLOUR('',#6295);
#6297=FILL_AREA_STYLE('',(#6296));
#6298=SURFACE_STYLE_FILL_AREA(#6297);
#6299=SURFACE_SIDE_STYLE('',(#6298));
#6300=SURFACE_STYLE_USAGE(.BOTH.,#6299);
#6301=PRESENTATION_STYLE_ASSIGNMENT((#6300));
ENDSEC;
END-ISO-10303-21;
